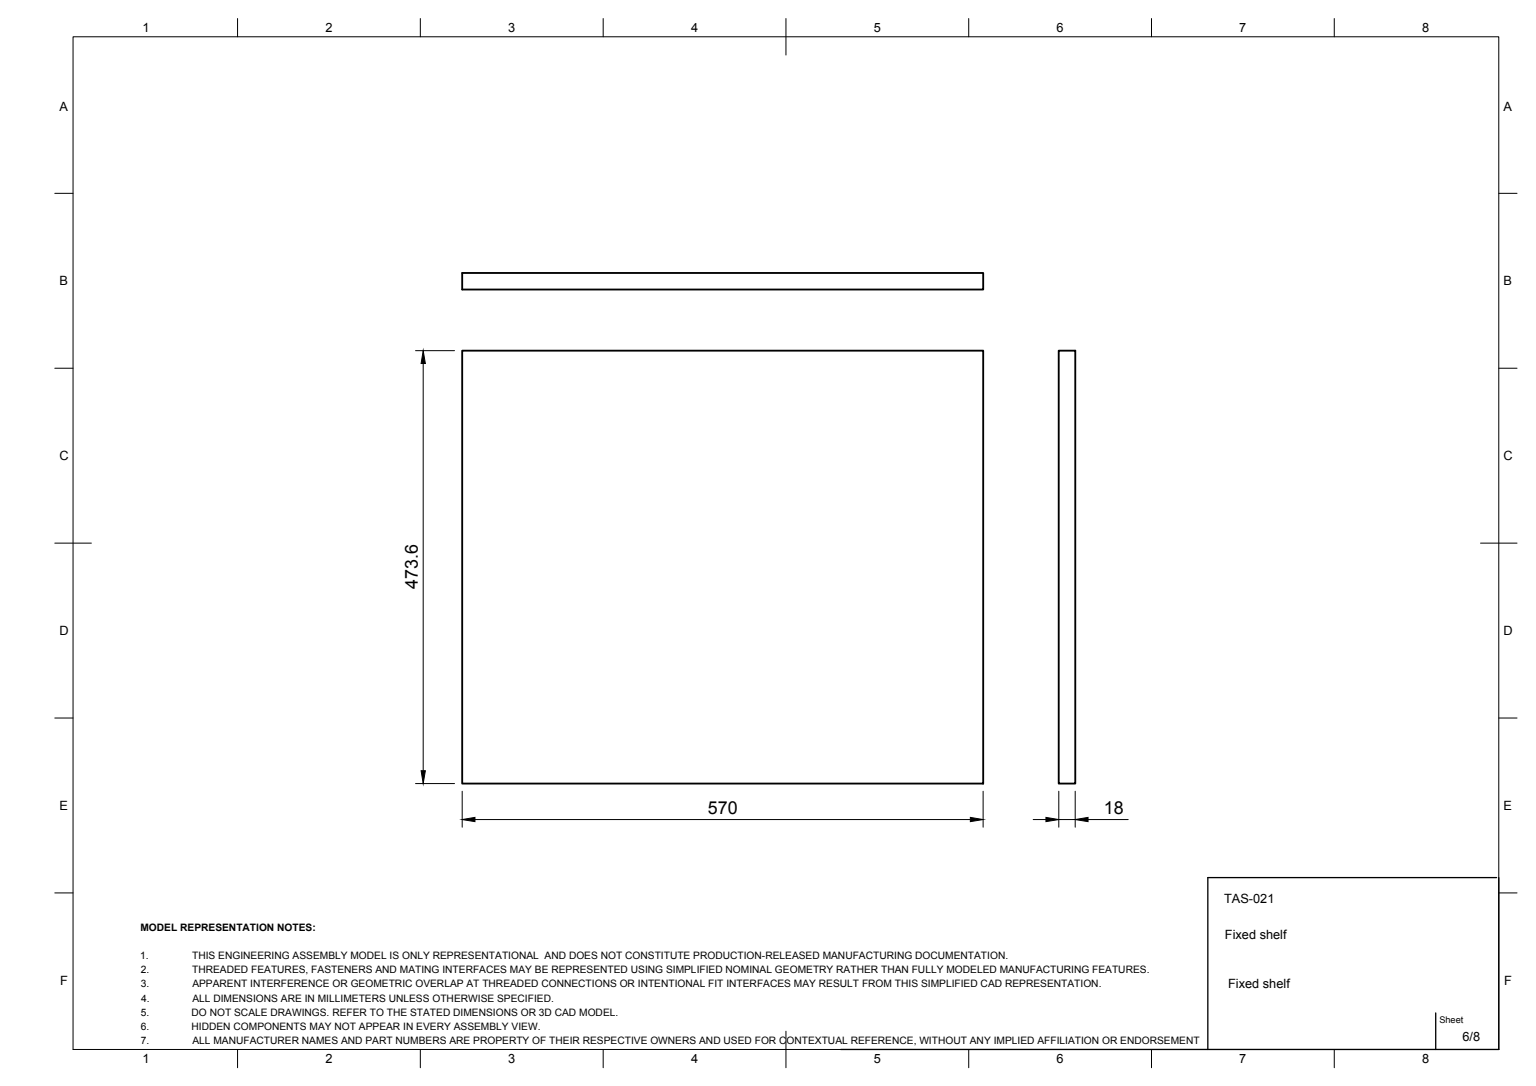
ISO-10303-21;
HEADER;
/* Generated by software containing ST-Developer
 * from STEP Tools, Inc. (www.steptools.com) 
 */

FILE_DESCRIPTION(
/* description */ (''),
/* implementation_level */ '2;1');

FILE_NAME(
/* name */ 'Fixed shelf.step',
/* time_stamp */ '2026-11-15T17:48:08-08:00',
/* author */ (''),
/* organization */ (''),
/* preprocessor_version */ 'ST-DEVELOPER v20.2',
/* originating_system */ 'Autodesk Translation Framework v15.17.0.0',
/* authorisation */ '');

FILE_SCHEMA (('AUTOMOTIVE_DESIGN { 1 0 10303 214 3 1 1 }'));
ENDSEC;

DATA;
#10=MECHANICAL_DESIGN_GEOMETRIC_PRESENTATION_REPRESENTATION('',(#142),#2097);
#130=SHAPE_REPRESENTATION_RELATIONSHIP('SRR','None',#2149,#136);
#136=ADVANCED_BREP_SHAPE_REPRESENTATION('',(#148),#2094);
#142=STYLED_ITEM('',(#2188),#148);
#148=MANIFOLD_SOLID_BREP('Body1',#1196);
#203=PLANE('',#1333);
#204=PLANE('',#1334);
#205=PLANE('',#1335);
#206=PLANE('',#1336);
#207=PLANE('',#1337);
#208=PLANE('',#1338);
#265=FACE_OUTER_BOUND('',#337,.T.);
#266=FACE_OUTER_BOUND('',#338,.T.);
#267=FACE_OUTER_BOUND('',#339,.T.);
#268=FACE_OUTER_BOUND('',#340,.T.);
#269=FACE_OUTER_BOUND('',#341,.T.);
#270=FACE_OUTER_BOUND('',#342,.T.);
#337=EDGE_LOOP('',(#1069,#1070,#1071,#1072));
#338=EDGE_LOOP('',(#1073,#1074,#1075,#1076));
#339=EDGE_LOOP('',(#1077,#1078,#1079,#1080));
#340=EDGE_LOOP('',(#1081,#1082,#1083,#1084));
#341=EDGE_LOOP('',(#1085,#1086,#1087,#1088));
#342=EDGE_LOOP('',(#1089,#1090,#1091,#1092));
#457=LINE('',#1998,#575);
#458=LINE('',#2000,#576);
#459=LINE('',#2002,#577);
#460=LINE('',#2003,#578);
#461=LINE('',#2006,#579);
#462=LINE('',#2008,#580);
#463=LINE('',#2009,#581);
#464=LINE('',#2012,#582);
#465=LINE('',#2014,#583);
#466=LINE('',#2015,#584);
#467=LINE('',#2017,#585);
#468=LINE('',#2018,#586);
#575=VECTOR('',#1626,1.);
#576=VECTOR('',#1627,1.);
#577=VECTOR('',#1628,1.);
#578=VECTOR('',#1629,1.);
#579=VECTOR('',#1632,1.);
#580=VECTOR('',#1633,1.);
#581=VECTOR('',#1634,1.);
#582=VECTOR('',#1637,1.);
#583=VECTOR('',#1638,1.);
#584=VECTOR('',#1639,1.);
#585=VECTOR('',#1642,1.);
#586=VECTOR('',#1643,1.);
#687=VERTEX_POINT('',#1996);
#688=VERTEX_POINT('',#1997);
#689=VERTEX_POINT('',#1999);
#690=VERTEX_POINT('',#2001);
#691=VERTEX_POINT('',#2005);
#692=VERTEX_POINT('',#2007);
#693=VERTEX_POINT('',#2011);
#694=VERTEX_POINT('',#2013);
#817=EDGE_CURVE('',#687,#688,#457,.T.);
#818=EDGE_CURVE('',#688,#689,#458,.T.);
#819=EDGE_CURVE('',#690,#689,#459,.T.);
#820=EDGE_CURVE('',#687,#690,#460,.T.);
#821=EDGE_CURVE('',#691,#687,#461,.T.);
#822=EDGE_CURVE('',#692,#690,#462,.T.);
#823=EDGE_CURVE('',#691,#692,#463,.T.);
#824=EDGE_CURVE('',#693,#691,#464,.T.);
#825=EDGE_CURVE('',#694,#692,#465,.T.);
#826=EDGE_CURVE('',#693,#694,#466,.T.);
#827=EDGE_CURVE('',#688,#693,#467,.T.);
#828=EDGE_CURVE('',#689,#694,#468,.T.);
#1069=ORIENTED_EDGE('',*,*,#817,.T.);
#1070=ORIENTED_EDGE('',*,*,#818,.T.);
#1071=ORIENTED_EDGE('',*,*,#819,.F.);
#1072=ORIENTED_EDGE('',*,*,#820,.F.);
#1073=ORIENTED_EDGE('',*,*,#821,.T.);
#1074=ORIENTED_EDGE('',*,*,#820,.T.);
#1075=ORIENTED_EDGE('',*,*,#822,.F.);
#1076=ORIENTED_EDGE('',*,*,#823,.F.);
#1077=ORIENTED_EDGE('',*,*,#824,.T.);
#1078=ORIENTED_EDGE('',*,*,#823,.T.);
#1079=ORIENTED_EDGE('',*,*,#825,.F.);
#1080=ORIENTED_EDGE('',*,*,#826,.F.);
#1081=ORIENTED_EDGE('',*,*,#827,.T.);
#1082=ORIENTED_EDGE('',*,*,#826,.T.);
#1083=ORIENTED_EDGE('',*,*,#828,.F.);
#1084=ORIENTED_EDGE('',*,*,#818,.F.);
#1085=ORIENTED_EDGE('',*,*,#828,.T.);
#1086=ORIENTED_EDGE('',*,*,#825,.T.);
#1087=ORIENTED_EDGE('',*,*,#822,.T.);
#1088=ORIENTED_EDGE('',*,*,#819,.T.);
#1089=ORIENTED_EDGE('',*,*,#827,.F.);
#1090=ORIENTED_EDGE('',*,*,#817,.F.);
#1091=ORIENTED_EDGE('',*,*,#821,.F.);
#1092=ORIENTED_EDGE('',*,*,#824,.F.);
#1177=ADVANCED_FACE('',(#265),#203,.T.);
#1178=ADVANCED_FACE('',(#266),#204,.T.);
#1179=ADVANCED_FACE('',(#267),#205,.T.);
#1180=ADVANCED_FACE('',(#268),#206,.T.);
#1181=ADVANCED_FACE('',(#269),#207,.T.);
#1182=ADVANCED_FACE('',(#270),#208,.F.);
#1196=CLOSED_SHELL('',(#1177,#1178,#1179,#1180,#1181,#1182));
#1332=AXIS2_PLACEMENT_3D('',#1994,#1622,#1623);
#1333=AXIS2_PLACEMENT_3D('',#1995,#1624,#1625);
#1334=AXIS2_PLACEMENT_3D('',#2004,#1630,#1631);
#1335=AXIS2_PLACEMENT_3D('',#2010,#1635,#1636);
#1336=AXIS2_PLACEMENT_3D('',#2016,#1640,#1641);
#1337=AXIS2_PLACEMENT_3D('',#2019,#1644,#1645);
#1338=AXIS2_PLACEMENT_3D('',#2020,#1646,#1647);
#1622=DIRECTION('axis',(0.,0.,1.));
#1623=DIRECTION('refdir',(1.,0.,0.));
#1624=DIRECTION('center_axis',(0.,1.,0.));
#1625=DIRECTION('ref_axis',(-1.,0.,0.));
#1626=DIRECTION('',(-1.,0.,0.));
#1627=DIRECTION('',(0.,0.,1.));
#1628=DIRECTION('',(-1.,0.,0.));
#1629=DIRECTION('',(0.,0.,1.));
#1630=DIRECTION('center_axis',(1.,0.,0.));
#1631=DIRECTION('ref_axis',(0.,1.,0.));
#1632=DIRECTION('',(0.,1.,0.));
#1633=DIRECTION('',(0.,1.,0.));
#1634=DIRECTION('',(0.,0.,1.));
#1635=DIRECTION('center_axis',(0.,-1.,0.));
#1636=DIRECTION('ref_axis',(1.,0.,0.));
#1637=DIRECTION('',(1.,0.,0.));
#1638=DIRECTION('',(1.,0.,0.));
#1639=DIRECTION('',(0.,0.,1.));
#1640=DIRECTION('center_axis',(-1.,0.,0.));
#1641=DIRECTION('ref_axis',(0.,-1.,0.));
#1642=DIRECTION('',(0.,-1.,0.));
#1643=DIRECTION('',(0.,-1.,0.));
#1644=DIRECTION('center_axis',(0.,0.,1.));
#1645=DIRECTION('ref_axis',(1.,0.,0.));
#1646=DIRECTION('center_axis',(0.,0.,1.));
#1647=DIRECTION('ref_axis',(1.,0.,0.));
#1994=CARTESIAN_POINT('',(0.,0.,0.));
#1995=CARTESIAN_POINT('Origin',(47.36,57.6,0.));
#1996=CARTESIAN_POINT('',(47.36,57.6,0.));
#1997=CARTESIAN_POINT('',(0.,57.6,0.));
#1998=CARTESIAN_POINT('',(47.36,57.6,0.));
#1999=CARTESIAN_POINT('',(0.,57.6,1.8));
#2000=CARTESIAN_POINT('',(0.,57.6,0.));
#2001=CARTESIAN_POINT('',(47.36,57.6,1.8));
#2002=CARTESIAN_POINT('',(47.36,57.6,1.8));
#2003=CARTESIAN_POINT('',(47.36,57.6,0.));
#2004=CARTESIAN_POINT('Origin',(47.36,0.6,0.));
#2005=CARTESIAN_POINT('',(47.36,0.6,0.));
#2006=CARTESIAN_POINT('',(47.36,0.6,0.));
#2007=CARTESIAN_POINT('',(47.36,0.600000000000001,1.8));
#2008=CARTESIAN_POINT('',(47.36,0.6,1.8));
#2009=CARTESIAN_POINT('',(47.36,0.6,0.));
#2010=CARTESIAN_POINT('Origin',(0.,0.6,0.));
#2011=CARTESIAN_POINT('',(0.,0.600000000000001,0.));
#2012=CARTESIAN_POINT('',(0.,0.6,0.));
#2013=CARTESIAN_POINT('',(0.,0.600000000000001,1.8));
#2014=CARTESIAN_POINT('',(0.,0.6,1.8));
#2015=CARTESIAN_POINT('',(0.,0.600000000000001,0.));
#2016=CARTESIAN_POINT('Origin',(0.,57.6,0.));
#2017=CARTESIAN_POINT('',(0.,57.6,0.));
#2018=CARTESIAN_POINT('',(0.,57.6,1.8));
#2019=CARTESIAN_POINT('Origin',(23.68,29.1,1.8));
#2020=CARTESIAN_POINT('Origin',(23.68,29.1,0.));
#2086=UNCERTAINTY_MEASURE_WITH_UNIT(LENGTH_MEASURE(0.001),#2098,
'DISTANCE_ACCURACY_VALUE',
'Maximum model space distance between geometric entities at asserted c
onnectivities');
#2089=UNCERTAINTY_MEASURE_WITH_UNIT(LENGTH_MEASURE(0.001),#2098,
'DISTANCE_ACCURACY_VALUE',
'Maximum model space distance between geometric entities at asserted c
onnectivities');
#2094=(
GEOMETRIC_REPRESENTATION_CONTEXT(3)
GLOBAL_UNCERTAINTY_ASSIGNED_CONTEXT((#2086))
GLOBAL_UNIT_ASSIGNED_CONTEXT((#2098,#2100,#2101))
REPRESENTATION_CONTEXT('','3D')
);
#2097=(
GEOMETRIC_REPRESENTATION_CONTEXT(3)
GLOBAL_UNCERTAINTY_ASSIGNED_CONTEXT((#2089))
GLOBAL_UNIT_ASSIGNED_CONTEXT((#2098,#2100,#2101))
REPRESENTATION_CONTEXT('','3D')
);
#2098=(
LENGTH_UNIT()
NAMED_UNIT(*)
SI_UNIT(.CENTI.,.METRE.)
);
#2100=(
NAMED_UNIT(*)
PLANE_ANGLE_UNIT()
SI_UNIT($,.RADIAN.)
);
#2101=(
NAMED_UNIT(*)
SI_UNIT($,.STERADIAN.)
SOLID_ANGLE_UNIT()
);
#2106=SHAPE_DEFINITION_REPRESENTATION(#2113,#2149);
#2113=PRODUCT_DEFINITION_SHAPE('',$,#2157);
#2149=SHAPE_REPRESENTATION('',(#1332),#2094);
#2152=PRODUCT_DEFINITION_CONTEXT('part definition',#2175,'design');
#2157=PRODUCT_DEFINITION('Fixed shelf','Fixed shelf',#2164,#2152);
#2164=PRODUCT_DEFINITION_FORMATION('',$,#2181);
#2175=APPLICATION_CONTEXT(
'Core Data for Automotive Mechanical Design Process');
#2176=PRODUCT_CONTEXT('part definition',#2175,'mechanical');
#2181=PRODUCT('Fixed shelf','Fixed shelf',$,(#2176));
#2188=PRESENTATION_STYLE_ASSIGNMENT((#2195));
#2195=SURFACE_STYLE_USAGE(.BOTH.,#2202);
#2202=SURFACE_SIDE_STYLE('',(#2209));
#2209=SURFACE_STYLE_FILL_AREA(#2216);
#2216=FILL_AREA_STYLE('Fixed shelf finish',(#2223));
#2223=FILL_AREA_STYLE_COLOUR('Fixed shelf finish',#2230);
#2230=COLOUR_RGB('Fixed shelf finish',0.274509803921569,0.6,0.8);
ENDSEC;
END-ISO-10303-21;
